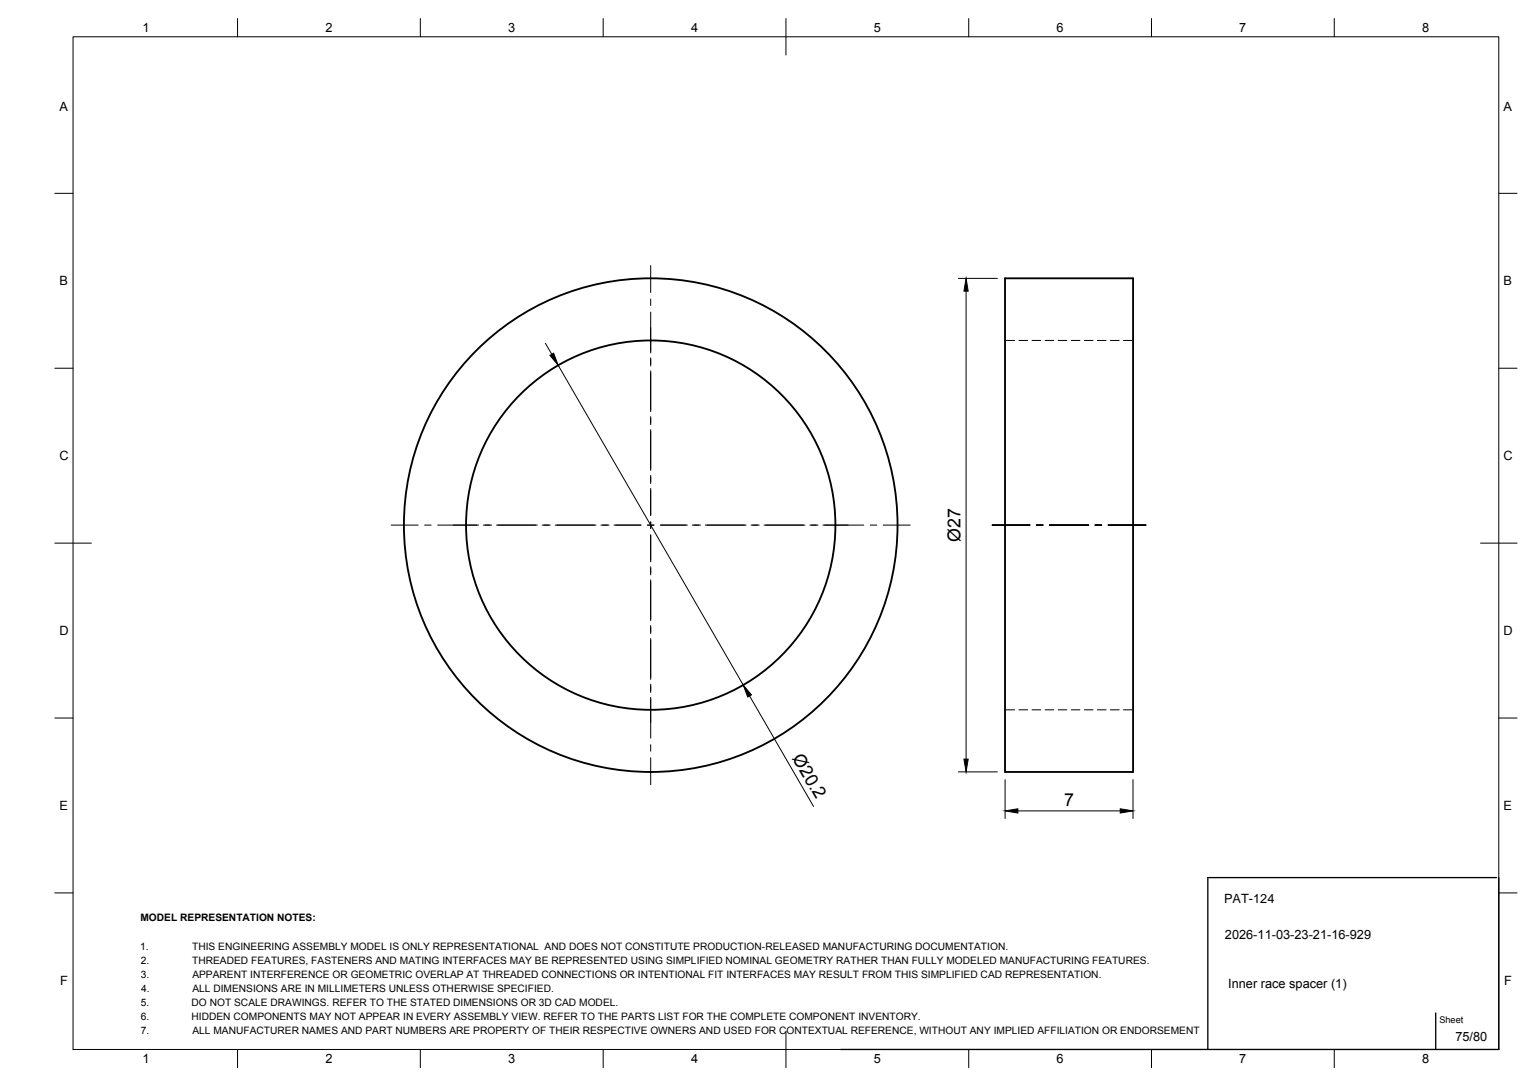
ISO-10303-21;
HEADER;
/* Generated by software containing ST-Developer
 * from STEP Tools, Inc. (www.steptools.com) 
 */

FILE_DESCRIPTION(
/* description */ ('XY cross-slide table'),
/* implementation_level */ '2;1');

FILE_NAME(
/* name */ 'Inner race spacer (1).step',
/* time_stamp */ '2026-10-28T03:22:46-07:00',
/* author */ (''),
/* organization */ (''),
/* preprocessor_version */ 'ST-DEVELOPER v20.2',
/* originating_system */ 'Autodesk Translation Framework v15.17.0.0',
/* authorisation */ '');

FILE_SCHEMA (('AUTOMOTIVE_DESIGN { 1 0 10303 214 3 1 1 }'));
ENDSEC;

DATA;
#10=MECHANICAL_DESIGN_GEOMETRIC_PRESENTATION_REPRESENTATION('',(#1774),#62984);
#1578=SHAPE_REPRESENTATION_RELATIONSHIP('SRR','None',#63438,#1661);
#1661=ADVANCED_BREP_SHAPE_REPRESENTATION('',(#1879),#62975);
#1774=STYLED_ITEM('',(#63912),#1879);
#1879=MANIFOLD_SOLID_BREP('Body1',#23076);
#2276=FACE_BOUND('',#5814,.T.);
#2277=FACE_BOUND('',#5816,.T.);
#2819=PLANE('',#26289);
#2820=PLANE('',#26290);
#4108=FACE_OUTER_BOUND('',#5811,.T.);
#4109=FACE_OUTER_BOUND('',#5812,.T.);
#4110=FACE_OUTER_BOUND('',#5813,.T.);
#4111=FACE_OUTER_BOUND('',#5815,.T.);
#5811=EDGE_LOOP('',(#20730,#20731,#20732,#20733));
#5812=EDGE_LOOP('',(#20734,#20735,#20736,#20737));
#5813=EDGE_LOOP('',(#20738));
#5814=EDGE_LOOP('',(#20739));
#5815=EDGE_LOOP('',(#20740));
#5816=EDGE_LOOP('',(#20741));
#7292=LINE('',#62286,#8779);
#7293=LINE('',#62292,#8780);
#8779=VECTOR('',#32417,1.01);
#8780=VECTOR('',#32424,1.35);
#9729=CIRCLE('',#26284,1.01);
#9730=CIRCLE('',#26285,1.01);
#9731=CIRCLE('',#26287,1.35);
#9732=CIRCLE('',#26288,1.35);
#11734=VERTEX_POINT('',#62283);
#11735=VERTEX_POINT('',#62285);
#11736=VERTEX_POINT('',#62289);
#11737=VERTEX_POINT('',#62291);
#14749=EDGE_CURVE('',#11734,#11734,#9729,.T.);
#14750=EDGE_CURVE('',#11734,#11735,#7292,.T.);
#14751=EDGE_CURVE('',#11735,#11735,#9730,.T.);
#14752=EDGE_CURVE('',#11736,#11736,#9731,.T.);
#14753=EDGE_CURVE('',#11736,#11737,#7293,.T.);
#14754=EDGE_CURVE('',#11737,#11737,#9732,.T.);
#20730=ORIENTED_EDGE('',*,*,#14749,.F.);
#20731=ORIENTED_EDGE('',*,*,#14750,.T.);
#20732=ORIENTED_EDGE('',*,*,#14751,.T.);
#20733=ORIENTED_EDGE('',*,*,#14750,.F.);
#20734=ORIENTED_EDGE('',*,*,#14752,.F.);
#20735=ORIENTED_EDGE('',*,*,#14753,.T.);
#20736=ORIENTED_EDGE('',*,*,#14754,.T.);
#20737=ORIENTED_EDGE('',*,*,#14753,.F.);
#20738=ORIENTED_EDGE('',*,*,#14752,.T.);
#20739=ORIENTED_EDGE('',*,*,#14749,.T.);
#20740=ORIENTED_EDGE('',*,*,#14754,.F.);
#20741=ORIENTED_EDGE('',*,*,#14751,.F.);
#21631=CYLINDRICAL_SURFACE('',#26283,1.01);
#21632=CYLINDRICAL_SURFACE('',#26286,1.35);
#22889=ADVANCED_FACE('',(#4108),#21631,.F.);
#22890=ADVANCED_FACE('',(#4109),#21632,.T.);
#22891=ADVANCED_FACE('',(#4110,#2276),#2819,.T.);
#22892=ADVANCED_FACE('',(#4111,#2277),#2820,.F.);
#23076=CLOSED_SHELL('',(#22889,#22890,#22891,#22892));
#26282=AXIS2_PLACEMENT_3D('',#62281,#32411,#32412);
#26283=AXIS2_PLACEMENT_3D('',#62282,#32413,#32414);
#26284=AXIS2_PLACEMENT_3D('',#62284,#32415,#32416);
#26285=AXIS2_PLACEMENT_3D('',#62287,#32418,#32419);
#26286=AXIS2_PLACEMENT_3D('',#62288,#32420,#32421);
#26287=AXIS2_PLACEMENT_3D('',#62290,#32422,#32423);
#26288=AXIS2_PLACEMENT_3D('',#62293,#32425,#32426);
#26289=AXIS2_PLACEMENT_3D('',#62294,#32427,#32428);
#26290=AXIS2_PLACEMENT_3D('',#62295,#32429,#32430);
#32411=DIRECTION('axis',(0.,0.,1.));
#32412=DIRECTION('refdir',(1.,0.,0.));
#32413=DIRECTION('center_axis',(1.,0.,0.));
#32414=DIRECTION('ref_axis',(0.,0.,-1.));
#32415=DIRECTION('center_axis',(-1.,0.,0.));
#32416=DIRECTION('ref_axis',(0.,0.,-1.));
#32417=DIRECTION('',(-1.,0.,0.));
#32418=DIRECTION('center_axis',(-1.,0.,0.));
#32419=DIRECTION('ref_axis',(0.,0.,-1.));
#32420=DIRECTION('center_axis',(1.,0.,0.));
#32421=DIRECTION('ref_axis',(0.,0.,-1.));
#32422=DIRECTION('center_axis',(1.,0.,0.));
#32423=DIRECTION('ref_axis',(0.,0.,-1.));
#32424=DIRECTION('',(-1.,0.,0.));
#32425=DIRECTION('center_axis',(1.,0.,0.));
#32426=DIRECTION('ref_axis',(0.,0.,-1.));
#32427=DIRECTION('center_axis',(1.,0.,0.));
#32428=DIRECTION('ref_axis',(0.,0.,-1.));
#32429=DIRECTION('center_axis',(1.,0.,0.));
#32430=DIRECTION('ref_axis',(0.,0.,-1.));
#62281=CARTESIAN_POINT('',(0.,0.,0.));
#62282=CARTESIAN_POINT('Origin',(24.7,0.,4.));
#62283=CARTESIAN_POINT('',(25.4,-1.23689326713883E-16,5.01));
#62284=CARTESIAN_POINT('Origin',(25.4,0.,4.));
#62285=CARTESIAN_POINT('',(24.7,-1.23689326713883E-16,5.01));
#62286=CARTESIAN_POINT('',(24.7,-1.23689326713883E-16,5.01));
#62287=CARTESIAN_POINT('Origin',(24.7,0.,4.));
#62288=CARTESIAN_POINT('Origin',(24.7,0.,4.));
#62289=CARTESIAN_POINT('',(25.4,-1.65327317884893E-16,5.35));
#62290=CARTESIAN_POINT('Origin',(25.4,0.,4.));
#62291=CARTESIAN_POINT('',(24.7,-1.65327317884893E-16,5.35));
#62292=CARTESIAN_POINT('',(24.7,-1.65327317884893E-16,5.35));
#62293=CARTESIAN_POINT('Origin',(24.7,0.,4.));
#62294=CARTESIAN_POINT('Origin',(25.4,0.,4.));
#62295=CARTESIAN_POINT('Origin',(24.7,0.,4.));
#62876=UNCERTAINTY_MEASURE_WITH_UNIT(LENGTH_MEASURE(0.001),#62985,
'DISTANCE_ACCURACY_VALUE',
'Maximum model space distance between geometric entities at asserted c
onnectivities');
#62885=UNCERTAINTY_MEASURE_WITH_UNIT(LENGTH_MEASURE(0.001),#62985,
'DISTANCE_ACCURACY_VALUE',
'Maximum model space distance between geometric entities at asserted c
onnectivities');
#62975=(
GEOMETRIC_REPRESENTATION_CONTEXT(3)
GLOBAL_UNCERTAINTY_ASSIGNED_CONTEXT((#62876))
GLOBAL_UNIT_ASSIGNED_CONTEXT((#62985,#62987,#62988))
REPRESENTATION_CONTEXT('','3D')
);
#62984=(
GEOMETRIC_REPRESENTATION_CONTEXT(3)
GLOBAL_UNCERTAINTY_ASSIGNED_CONTEXT((#62885))
GLOBAL_UNIT_ASSIGNED_CONTEXT((#62985,#62987,#62988))
REPRESENTATION_CONTEXT('','3D')
);
#62985=(
LENGTH_UNIT()
NAMED_UNIT(*)
SI_UNIT(.CENTI.,.METRE.)
);
#62987=(
NAMED_UNIT(*)
PLANE_ANGLE_UNIT()
SI_UNIT($,.RADIAN.)
);
#62988=(
NAMED_UNIT(*)
SI_UNIT($,.STERADIAN.)
SOLID_ANGLE_UNIT()
);
#63078=SHAPE_DEFINITION_REPRESENTATION(#63289,#63438);
#63289=PRODUCT_DEFINITION_SHAPE('',$,#63537);
#63438=SHAPE_REPRESENTATION('',(#26282),#62975);
#63447=PRODUCT_DEFINITION_CONTEXT('part definition',#63743,'design');
#63537=PRODUCT_DEFINITION('Inner race spacer (1)','Inner race spacer (1)',
#63635,#63447);
#63635=PRODUCT_DEFINITION_FORMATION('',$,#63834);
#63743=APPLICATION_CONTEXT(
'Core Data for Automotive Mechanical Design Process');
#63744=PRODUCT_CONTEXT('part definition',#63743,'mechanical');
#63834=PRODUCT('Inner race spacer (1)','Inner race spacer (1)',
'Inner race spacer (1)',(#63744));
#63906=COLOUR_RGB('Grey',0.48,0.52,0.57);
#63907=FILL_AREA_STYLE_COLOUR('',#63906);
#63908=FILL_AREA_STYLE('',(#63907));
#63909=SURFACE_STYLE_FILL_AREA(#63908);
#63910=SURFACE_SIDE_STYLE('',(#63909));
#63911=SURFACE_STYLE_USAGE(.BOTH.,#63910);
#63912=PRESENTATION_STYLE_ASSIGNMENT((#63911));
ENDSEC;
END-ISO-10303-21;
